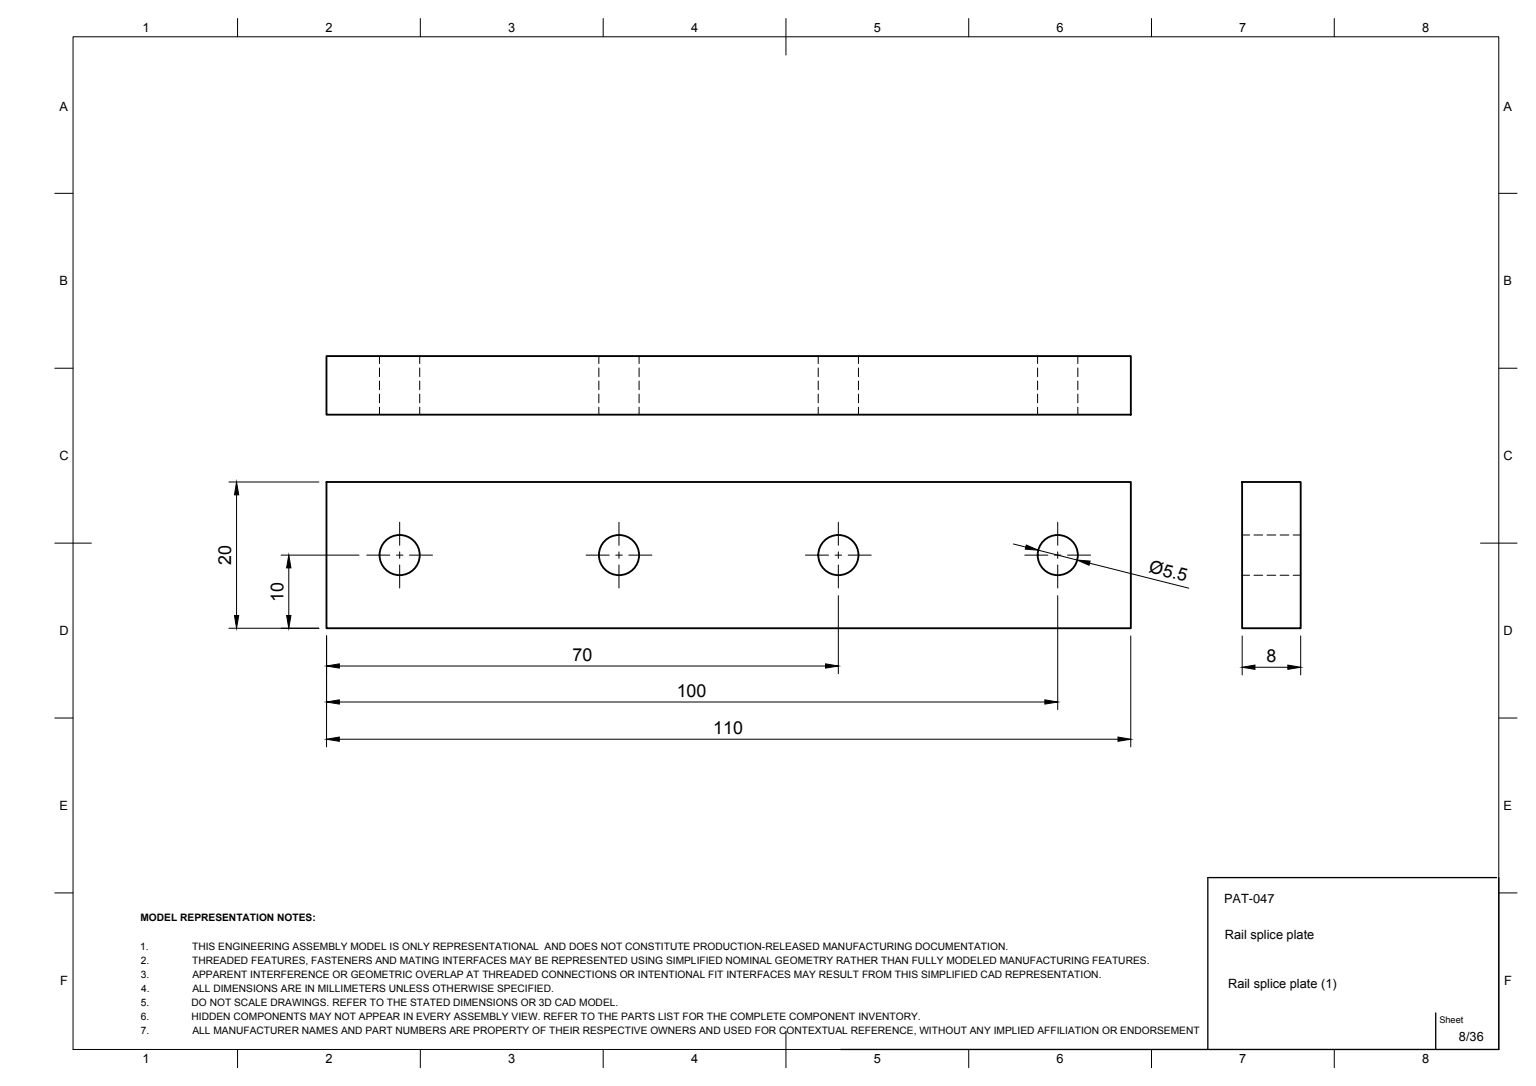
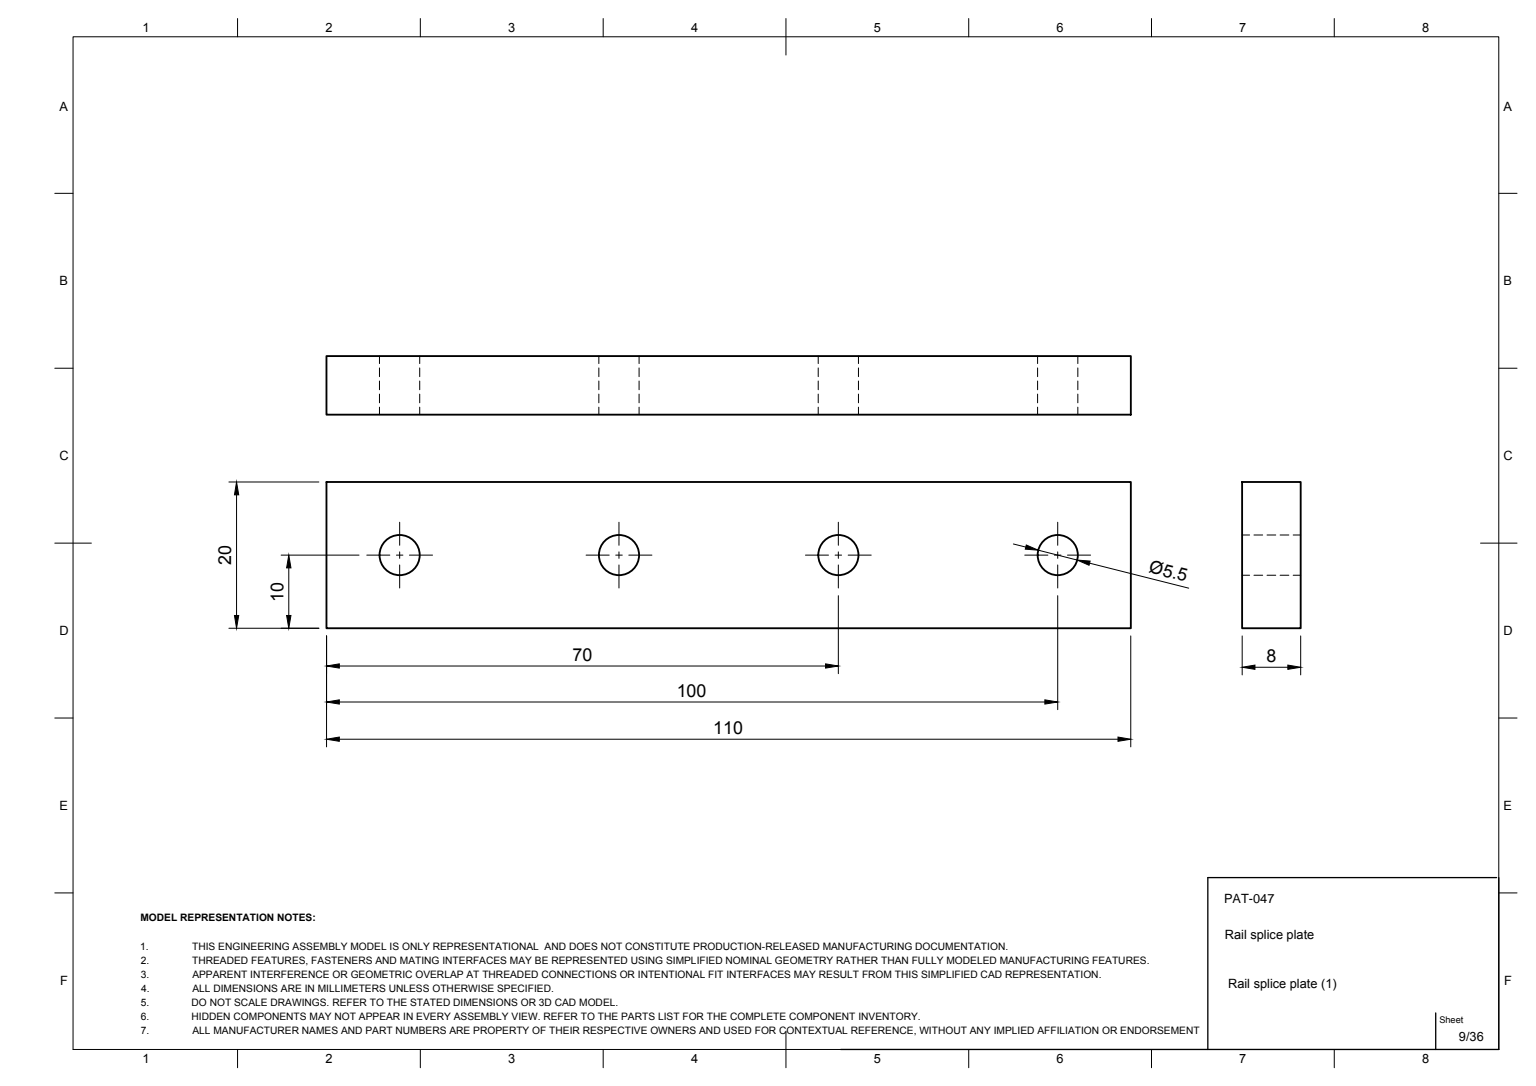
ISO-10303-21;
HEADER;
/* Generated by software containing ST-Developer
 * from STEP Tools, Inc. (www.steptools.com) 
 */

FILE_DESCRIPTION(
/* description */ ('Gravity roller conveyor section'),
/* implementation_level */ '2;1');

FILE_NAME(
/* name */ 'Rail splice plate (1).step',
/* time_stamp */ '2026-11-02T07:43:02-08:00',
/* author */ (''),
/* organization */ (''),
/* preprocessor_version */ 'ST-DEVELOPER v20.2',
/* originating_system */ 'Autodesk Translation Framework v15.17.0.0',
/* authorisation */ '');

FILE_SCHEMA (('AUTOMOTIVE_DESIGN { 1 0 10303 214 3 1 1 }'));
ENDSEC;

DATA;
#10=MECHANICAL_DESIGN_GEOMETRIC_PRESENTATION_REPRESENTATION('',(#535),#13821);
#467=SHAPE_REPRESENTATION_RELATIONSHIP('SRR','None',#14004,#501);
#501=ADVANCED_BREP_SHAPE_REPRESENTATION('',(#575),#13791);
#535=STYLED_ITEM('',(#14191),#575);
#575=MANIFOLD_SOLID_BREP('Body1',#7635);
#632=FACE_BOUND('',#1644,.T.);
#633=FACE_BOUND('',#1645,.T.);
#634=FACE_BOUND('',#1646,.T.);
#635=FACE_BOUND('',#1647,.T.);
#636=FACE_BOUND('',#1650,.T.);
#637=FACE_BOUND('',#1651,.T.);
#638=FACE_BOUND('',#1652,.T.);
#639=FACE_BOUND('',#1653,.T.);
#869=PLANE('',#8294);
#870=PLANE('',#8295);
#871=PLANE('',#8296);
#872=PLANE('',#8297);
#873=PLANE('',#8298);
#874=PLANE('',#8299);
#1197=FACE_OUTER_BOUND('',#1639,.T.);
#1198=FACE_OUTER_BOUND('',#1640,.T.);
#1199=FACE_OUTER_BOUND('',#1641,.T.);
#1200=FACE_OUTER_BOUND('',#1642,.T.);
#1201=FACE_OUTER_BOUND('',#1643,.T.);
#1202=FACE_OUTER_BOUND('',#1648,.T.);
#1203=FACE_OUTER_BOUND('',#1649,.T.);
#1204=FACE_OUTER_BOUND('',#1654,.T.);
#1205=FACE_OUTER_BOUND('',#1655,.T.);
#1206=FACE_OUTER_BOUND('',#1656,.T.);
#1639=EDGE_LOOP('',(#6230,#6231,#6232,#6233));
#1640=EDGE_LOOP('',(#6234,#6235,#6236,#6237));
#1641=EDGE_LOOP('',(#6238,#6239,#6240,#6241));
#1642=EDGE_LOOP('',(#6242,#6243,#6244,#6245));
#1643=EDGE_LOOP('',(#6246,#6247,#6248,#6249));
#1644=EDGE_LOOP('',(#6250));
#1645=EDGE_LOOP('',(#6251));
#1646=EDGE_LOOP('',(#6252));
#1647=EDGE_LOOP('',(#6253));
#1648=EDGE_LOOP('',(#6254,#6255,#6256,#6257));
#1649=EDGE_LOOP('',(#6258,#6259,#6260,#6261));
#1650=EDGE_LOOP('',(#6262));
#1651=EDGE_LOOP('',(#6263));
#1652=EDGE_LOOP('',(#6264));
#1653=EDGE_LOOP('',(#6265));
#1654=EDGE_LOOP('',(#6266,#6267,#6268,#6269));
#1655=EDGE_LOOP('',(#6270,#6271,#6272,#6273));
#1656=EDGE_LOOP('',(#6274,#6275,#6276,#6277));
#2407=LINE('',#12301,#3125);
#2408=LINE('',#12307,#3126);
#2409=LINE('',#12313,#3127);
#2410=LINE('',#12319,#3128);
#2411=LINE('',#12324,#3129);
#2412=LINE('',#12326,#3130);
#2413=LINE('',#12328,#3131);
#2414=LINE('',#12329,#3132);
#2415=LINE('',#12332,#3133);
#2416=LINE('',#12334,#3134);
#2417=LINE('',#12335,#3135);
#2418=LINE('',#12338,#3136);
#2419=LINE('',#12340,#3137);
#2420=LINE('',#12341,#3138);
#2421=LINE('',#12343,#3139);
#2422=LINE('',#12344,#3140);
#3125=VECTOR('',#9758,0.274999999999999);
#3126=VECTOR('',#9765,0.274999999999999);
#3127=VECTOR('',#9772,0.274999999999999);
#3128=VECTOR('',#9779,0.274999999999999);
#3129=VECTOR('',#9784,1.);
#3130=VECTOR('',#9785,1.);
#3131=VECTOR('',#9786,1.);
#3132=VECTOR('',#9787,1.);
#3133=VECTOR('',#9790,1.);
#3134=VECTOR('',#9791,1.);
#3135=VECTOR('',#9792,1.);
#3136=VECTOR('',#9795,1.);
#3137=VECTOR('',#9796,1.);
#3138=VECTOR('',#9797,1.);
#3139=VECTOR('',#9800,1.);
#3140=VECTOR('',#9801,1.);
#3409=CIRCLE('',#8283,0.274999999999999);
#3410=CIRCLE('',#8284,0.274999999999999);
#3411=CIRCLE('',#8286,0.274999999999999);
#3412=CIRCLE('',#8287,0.274999999999999);
#3413=CIRCLE('',#8289,0.274999999999999);
#3414=CIRCLE('',#8290,0.274999999999999);
#3415=CIRCLE('',#8292,0.274999999999999);
#3416=CIRCLE('',#8293,0.274999999999999);
#3931=VERTEX_POINT('',#12298);
#3932=VERTEX_POINT('',#12300);
#3933=VERTEX_POINT('',#12304);
#3934=VERTEX_POINT('',#12306);
#3935=VERTEX_POINT('',#12310);
#3936=VERTEX_POINT('',#12312);
#3937=VERTEX_POINT('',#12316);
#3938=VERTEX_POINT('',#12318);
#3939=VERTEX_POINT('',#12322);
#3940=VERTEX_POINT('',#12323);
#3941=VERTEX_POINT('',#12325);
#3942=VERTEX_POINT('',#12327);
#3943=VERTEX_POINT('',#12331);
#3944=VERTEX_POINT('',#12333);
#3945=VERTEX_POINT('',#12337);
#3946=VERTEX_POINT('',#12339);
#4752=EDGE_CURVE('',#3931,#3931,#3409,.T.);
#4753=EDGE_CURVE('',#3931,#3932,#2407,.T.);
#4754=EDGE_CURVE('',#3932,#3932,#3410,.T.);
#4755=EDGE_CURVE('',#3933,#3933,#3411,.T.);
#4756=EDGE_CURVE('',#3933,#3934,#2408,.T.);
#4757=EDGE_CURVE('',#3934,#3934,#3412,.T.);
#4758=EDGE_CURVE('',#3935,#3935,#3413,.T.);
#4759=EDGE_CURVE('',#3935,#3936,#2409,.T.);
#4760=EDGE_CURVE('',#3936,#3936,#3414,.T.);
#4761=EDGE_CURVE('',#3937,#3937,#3415,.T.);
#4762=EDGE_CURVE('',#3937,#3938,#2410,.T.);
#4763=EDGE_CURVE('',#3938,#3938,#3416,.T.);
#4764=EDGE_CURVE('',#3939,#3940,#2411,.T.);
#4765=EDGE_CURVE('',#3940,#3941,#2412,.T.);
#4766=EDGE_CURVE('',#3942,#3941,#2413,.T.);
#4767=EDGE_CURVE('',#3939,#3942,#2414,.T.);
#4768=EDGE_CURVE('',#3943,#3939,#2415,.T.);
#4769=EDGE_CURVE('',#3944,#3942,#2416,.T.);
#4770=EDGE_CURVE('',#3943,#3944,#2417,.T.);
#4771=EDGE_CURVE('',#3945,#3943,#2418,.T.);
#4772=EDGE_CURVE('',#3946,#3944,#2419,.T.);
#4773=EDGE_CURVE('',#3945,#3946,#2420,.T.);
#4774=EDGE_CURVE('',#3940,#3945,#2421,.T.);
#4775=EDGE_CURVE('',#3941,#3946,#2422,.T.);
#6230=ORIENTED_EDGE('',*,*,#4752,.F.);
#6231=ORIENTED_EDGE('',*,*,#4753,.T.);
#6232=ORIENTED_EDGE('',*,*,#4754,.F.);
#6233=ORIENTED_EDGE('',*,*,#4753,.F.);
#6234=ORIENTED_EDGE('',*,*,#4755,.F.);
#6235=ORIENTED_EDGE('',*,*,#4756,.T.);
#6236=ORIENTED_EDGE('',*,*,#4757,.F.);
#6237=ORIENTED_EDGE('',*,*,#4756,.F.);
#6238=ORIENTED_EDGE('',*,*,#4758,.F.);
#6239=ORIENTED_EDGE('',*,*,#4759,.T.);
#6240=ORIENTED_EDGE('',*,*,#4760,.F.);
#6241=ORIENTED_EDGE('',*,*,#4759,.F.);
#6242=ORIENTED_EDGE('',*,*,#4761,.F.);
#6243=ORIENTED_EDGE('',*,*,#4762,.T.);
#6244=ORIENTED_EDGE('',*,*,#4763,.F.);
#6245=ORIENTED_EDGE('',*,*,#4762,.F.);
#6246=ORIENTED_EDGE('',*,*,#4764,.T.);
#6247=ORIENTED_EDGE('',*,*,#4765,.T.);
#6248=ORIENTED_EDGE('',*,*,#4766,.F.);
#6249=ORIENTED_EDGE('',*,*,#4767,.F.);
#6250=ORIENTED_EDGE('',*,*,#4754,.T.);
#6251=ORIENTED_EDGE('',*,*,#4757,.T.);
#6252=ORIENTED_EDGE('',*,*,#4760,.T.);
#6253=ORIENTED_EDGE('',*,*,#4763,.T.);
#6254=ORIENTED_EDGE('',*,*,#4768,.T.);
#6255=ORIENTED_EDGE('',*,*,#4767,.T.);
#6256=ORIENTED_EDGE('',*,*,#4769,.F.);
#6257=ORIENTED_EDGE('',*,*,#4770,.F.);
#6258=ORIENTED_EDGE('',*,*,#4771,.T.);
#6259=ORIENTED_EDGE('',*,*,#4770,.T.);
#6260=ORIENTED_EDGE('',*,*,#4772,.F.);
#6261=ORIENTED_EDGE('',*,*,#4773,.F.);
#6262=ORIENTED_EDGE('',*,*,#4752,.T.);
#6263=ORIENTED_EDGE('',*,*,#4755,.T.);
#6264=ORIENTED_EDGE('',*,*,#4758,.T.);
#6265=ORIENTED_EDGE('',*,*,#4761,.T.);
#6266=ORIENTED_EDGE('',*,*,#4774,.T.);
#6267=ORIENTED_EDGE('',*,*,#4773,.T.);
#6268=ORIENTED_EDGE('',*,*,#4775,.F.);
#6269=ORIENTED_EDGE('',*,*,#4765,.F.);
#6270=ORIENTED_EDGE('',*,*,#4775,.T.);
#6271=ORIENTED_EDGE('',*,*,#4772,.T.);
#6272=ORIENTED_EDGE('',*,*,#4769,.T.);
#6273=ORIENTED_EDGE('',*,*,#4766,.T.);
#6274=ORIENTED_EDGE('',*,*,#4774,.F.);
#6275=ORIENTED_EDGE('',*,*,#4764,.F.);
#6276=ORIENTED_EDGE('',*,*,#4768,.F.);
#6277=ORIENTED_EDGE('',*,*,#4771,.F.);
#7146=CYLINDRICAL_SURFACE('',#8282,0.274999999999999);
#7147=CYLINDRICAL_SURFACE('',#8285,0.274999999999999);
#7148=CYLINDRICAL_SURFACE('',#8288,0.274999999999999);
#7149=CYLINDRICAL_SURFACE('',#8291,0.274999999999999);
#7398=ADVANCED_FACE('',(#1197),#7146,.F.);
#7399=ADVANCED_FACE('',(#1198),#7147,.F.);
#7400=ADVANCED_FACE('',(#1199),#7148,.F.);
#7401=ADVANCED_FACE('',(#1200),#7149,.F.);
#7402=ADVANCED_FACE('',(#1201,#632,#633,#634,#635),#869,.T.);
#7403=ADVANCED_FACE('',(#1202),#870,.T.);
#7404=ADVANCED_FACE('',(#1203,#636,#637,#638,#639),#871,.T.);
#7405=ADVANCED_FACE('',(#1204),#872,.T.);
#7406=ADVANCED_FACE('',(#1205),#873,.T.);
#7407=ADVANCED_FACE('',(#1206),#874,.F.);
#7635=CLOSED_SHELL('',(#7398,#7399,#7400,#7401,#7402,#7403,#7404,#7405,
#7406,#7407));
#8281=AXIS2_PLACEMENT_3D('',#12296,#9752,#9753);
#8282=AXIS2_PLACEMENT_3D('',#12297,#9754,#9755);
#8283=AXIS2_PLACEMENT_3D('',#12299,#9756,#9757);
#8284=AXIS2_PLACEMENT_3D('',#12302,#9759,#9760);
#8285=AXIS2_PLACEMENT_3D('',#12303,#9761,#9762);
#8286=AXIS2_PLACEMENT_3D('',#12305,#9763,#9764);
#8287=AXIS2_PLACEMENT_3D('',#12308,#9766,#9767);
#8288=AXIS2_PLACEMENT_3D('',#12309,#9768,#9769);
#8289=AXIS2_PLACEMENT_3D('',#12311,#9770,#9771);
#8290=AXIS2_PLACEMENT_3D('',#12314,#9773,#9774);
#8291=AXIS2_PLACEMENT_3D('',#12315,#9775,#9776);
#8292=AXIS2_PLACEMENT_3D('',#12317,#9777,#9778);
#8293=AXIS2_PLACEMENT_3D('',#12320,#9780,#9781);
#8294=AXIS2_PLACEMENT_3D('',#12321,#9782,#9783);
#8295=AXIS2_PLACEMENT_3D('',#12330,#9788,#9789);
#8296=AXIS2_PLACEMENT_3D('',#12336,#9793,#9794);
#8297=AXIS2_PLACEMENT_3D('',#12342,#9798,#9799);
#8298=AXIS2_PLACEMENT_3D('',#12345,#9802,#9803);
#8299=AXIS2_PLACEMENT_3D('',#12346,#9804,#9805);
#9752=DIRECTION('axis',(0.,0.,1.));
#9753=DIRECTION('refdir',(1.,0.,0.));
#9754=DIRECTION('center_axis',(0.,1.,0.));
#9755=DIRECTION('ref_axis',(1.,0.,0.));
#9756=DIRECTION('center_axis',(0.,1.,0.));
#9757=DIRECTION('ref_axis',(1.,0.,0.));
#9758=DIRECTION('',(0.,1.,0.));
#9759=DIRECTION('center_axis',(0.,-1.,0.));
#9760=DIRECTION('ref_axis',(1.,0.,0.));
#9761=DIRECTION('center_axis',(0.,1.,0.));
#9762=DIRECTION('ref_axis',(1.,0.,0.));
#9763=DIRECTION('center_axis',(0.,1.,0.));
#9764=DIRECTION('ref_axis',(1.,0.,0.));
#9765=DIRECTION('',(0.,1.,0.));
#9766=DIRECTION('center_axis',(0.,-1.,0.));
#9767=DIRECTION('ref_axis',(1.,0.,0.));
#9768=DIRECTION('center_axis',(0.,1.,0.));
#9769=DIRECTION('ref_axis',(1.,0.,0.));
#9770=DIRECTION('center_axis',(0.,1.,0.));
#9771=DIRECTION('ref_axis',(1.,0.,0.));
#9772=DIRECTION('',(0.,1.,0.));
#9773=DIRECTION('center_axis',(0.,-1.,0.));
#9774=DIRECTION('ref_axis',(1.,0.,0.));
#9775=DIRECTION('center_axis',(0.,1.,0.));
#9776=DIRECTION('ref_axis',(1.,0.,0.));
#9777=DIRECTION('center_axis',(0.,1.,0.));
#9778=DIRECTION('ref_axis',(1.,0.,0.));
#9779=DIRECTION('',(0.,1.,0.));
#9780=DIRECTION('center_axis',(0.,-1.,0.));
#9781=DIRECTION('ref_axis',(1.,0.,0.));
#9782=DIRECTION('center_axis',(0.,1.,0.));
#9783=DIRECTION('ref_axis',(-1.,0.,0.));
#9784=DIRECTION('',(-1.,0.,0.));
#9785=DIRECTION('',(0.,0.,1.));
#9786=DIRECTION('',(-1.,0.,0.));
#9787=DIRECTION('',(0.,0.,1.));
#9788=DIRECTION('center_axis',(1.,0.,0.));
#9789=DIRECTION('ref_axis',(0.,1.,0.));
#9790=DIRECTION('',(0.,1.,0.));
#9791=DIRECTION('',(0.,1.,0.));
#9792=DIRECTION('',(0.,0.,1.));
#9793=DIRECTION('center_axis',(0.,-1.,0.));
#9794=DIRECTION('ref_axis',(1.,0.,0.));
#9795=DIRECTION('',(1.,0.,0.));
#9796=DIRECTION('',(1.,0.,0.));
#9797=DIRECTION('',(0.,0.,1.));
#9798=DIRECTION('center_axis',(-1.,0.,0.));
#9799=DIRECTION('ref_axis',(0.,-1.,0.));
#9800=DIRECTION('',(0.,-1.,0.));
#9801=DIRECTION('',(0.,-1.,0.));
#9802=DIRECTION('center_axis',(0.,0.,1.));
#9803=DIRECTION('ref_axis',(1.,0.,0.));
#9804=DIRECTION('center_axis',(0.,0.,1.));
#9805=DIRECTION('ref_axis',(1.,0.,0.));
#12296=CARTESIAN_POINT('',(0.,0.,0.));
#12297=CARTESIAN_POINT('Origin',(42.,30.1,5.));
#12298=CARTESIAN_POINT('',(41.725,33.,5.));
#12299=CARTESIAN_POINT('Origin',(42.,33.,5.));
#12300=CARTESIAN_POINT('',(41.725,33.8,5.));
#12301=CARTESIAN_POINT('',(41.725,30.1,5.));
#12302=CARTESIAN_POINT('Origin',(42.,33.8,5.));
#12303=CARTESIAN_POINT('Origin',(39.,30.1,5.));
#12304=CARTESIAN_POINT('',(38.725,33.,5.));
#12305=CARTESIAN_POINT('Origin',(39.,33.,5.));
#12306=CARTESIAN_POINT('',(38.725,33.8,5.));
#12307=CARTESIAN_POINT('',(38.725,30.1,5.));
#12308=CARTESIAN_POINT('Origin',(39.,33.8,5.));
#12309=CARTESIAN_POINT('Origin',(36.,30.1,5.));
#12310=CARTESIAN_POINT('',(35.725,33.,5.));
#12311=CARTESIAN_POINT('Origin',(36.,33.,5.));
#12312=CARTESIAN_POINT('',(35.725,33.8,5.));
#12313=CARTESIAN_POINT('',(35.725,30.1,5.));
#12314=CARTESIAN_POINT('Origin',(36.,33.8,5.));
#12315=CARTESIAN_POINT('Origin',(45.,30.1,5.));
#12316=CARTESIAN_POINT('',(44.725,33.,5.));
#12317=CARTESIAN_POINT('Origin',(45.,33.,5.));
#12318=CARTESIAN_POINT('',(44.725,33.8,5.));
#12319=CARTESIAN_POINT('',(44.725,30.1,5.));
#12320=CARTESIAN_POINT('Origin',(45.,33.8,5.));
#12321=CARTESIAN_POINT('Origin',(46.,33.8,4.));
#12322=CARTESIAN_POINT('',(46.,33.8,4.));
#12323=CARTESIAN_POINT('',(35.,33.8,4.));
#12324=CARTESIAN_POINT('',(46.,33.8,4.));
#12325=CARTESIAN_POINT('',(35.,33.8,6.));
#12326=CARTESIAN_POINT('',(35.,33.8,4.));
#12327=CARTESIAN_POINT('',(46.,33.8,6.));
#12328=CARTESIAN_POINT('',(46.,33.8,6.));
#12329=CARTESIAN_POINT('',(46.,33.8,4.));
#12330=CARTESIAN_POINT('Origin',(46.,33.,4.));
#12331=CARTESIAN_POINT('',(46.,33.,4.));
#12332=CARTESIAN_POINT('',(46.,33.,4.));
#12333=CARTESIAN_POINT('',(46.,33.,6.));
#12334=CARTESIAN_POINT('',(46.,33.,6.));
#12335=CARTESIAN_POINT('',(46.,33.,4.));
#12336=CARTESIAN_POINT('Origin',(35.,33.,4.));
#12337=CARTESIAN_POINT('',(35.,33.,4.));
#12338=CARTESIAN_POINT('',(35.,33.,4.));
#12339=CARTESIAN_POINT('',(35.,33.,6.));
#12340=CARTESIAN_POINT('',(35.,33.,6.));
#12341=CARTESIAN_POINT('',(35.,33.,4.));
#12342=CARTESIAN_POINT('Origin',(35.,33.8,4.));
#12343=CARTESIAN_POINT('',(35.,33.8,4.));
#12344=CARTESIAN_POINT('',(35.,33.8,6.));
#12345=CARTESIAN_POINT('Origin',(40.5,33.4,6.));
#12346=CARTESIAN_POINT('Origin',(40.5,33.4,4.));
#13752=UNCERTAINTY_MEASURE_WITH_UNIT(LENGTH_MEASURE(0.001),#13822,
'DISTANCE_ACCURACY_VALUE',
'Maximum model space distance between geometric entities at asserted c
onnectivities');
#13782=UNCERTAINTY_MEASURE_WITH_UNIT(LENGTH_MEASURE(0.001),#13822,
'DISTANCE_ACCURACY_VALUE',
'Maximum model space distance between geometric entities at asserted c
onnectivities');
#13791=(
GEOMETRIC_REPRESENTATION_CONTEXT(3)
GLOBAL_UNCERTAINTY_ASSIGNED_CONTEXT((#13752))
GLOBAL_UNIT_ASSIGNED_CONTEXT((#13822,#13824,#13825))
REPRESENTATION_CONTEXT('','3D')
);
#13821=(
GEOMETRIC_REPRESENTATION_CONTEXT(3)
GLOBAL_UNCERTAINTY_ASSIGNED_CONTEXT((#13782))
GLOBAL_UNIT_ASSIGNED_CONTEXT((#13822,#13824,#13825))
REPRESENTATION_CONTEXT('','3D')
);
#13822=(
LENGTH_UNIT()
NAMED_UNIT(*)
SI_UNIT(.CENTI.,.METRE.)
);
#13824=(
NAMED_UNIT(*)
PLANE_ANGLE_UNIT()
SI_UNIT($,.RADIAN.)
);
#13825=(
NAMED_UNIT(*)
SI_UNIT($,.STERADIAN.)
SOLID_ANGLE_UNIT()
);
#13834=SHAPE_DEFINITION_REPRESENTATION(#13872,#14004);
#13872=PRODUCT_DEFINITION_SHAPE('',$,#14043);
#14004=SHAPE_REPRESENTATION('',(#8281),#13791);
#14034=PRODUCT_DEFINITION_CONTEXT('part definition',#14150,'design');
#14043=PRODUCT_DEFINITION('Rail splice plate_1','Rail splice plate (1)',
#14081,#14034);
#14081=PRODUCT_DEFINITION_FORMATION('',$,#14160);
#14150=APPLICATION_CONTEXT(
'Core Data for Automotive Mechanical Design Process');
#14151=PRODUCT_CONTEXT('part definition',#14150,'mechanical');
#14160=PRODUCT('Rail splice plate_1','Rail splice plate (1)',
'Rail splice plate',(#14151));
#14191=PRESENTATION_STYLE_ASSIGNMENT((#14196));
#14196=SURFACE_STYLE_USAGE(.BOTH.,#14201);
#14201=SURFACE_SIDE_STYLE('',(#14206));
#14206=SURFACE_STYLE_FILL_AREA(#14211);
#14211=FILL_AREA_STYLE('CAD Library Painted - Steel gray',(#14216));
#14216=FILL_AREA_STYLE_COLOUR('CAD Library Painted - Steel gray',#14221);
#14221=COLOUR_RGB('CAD Library Painted - Steel gray',0.592156862745098,
0.631372549019608,0.67843137254902);
ENDSEC;
END-ISO-10303-21;
